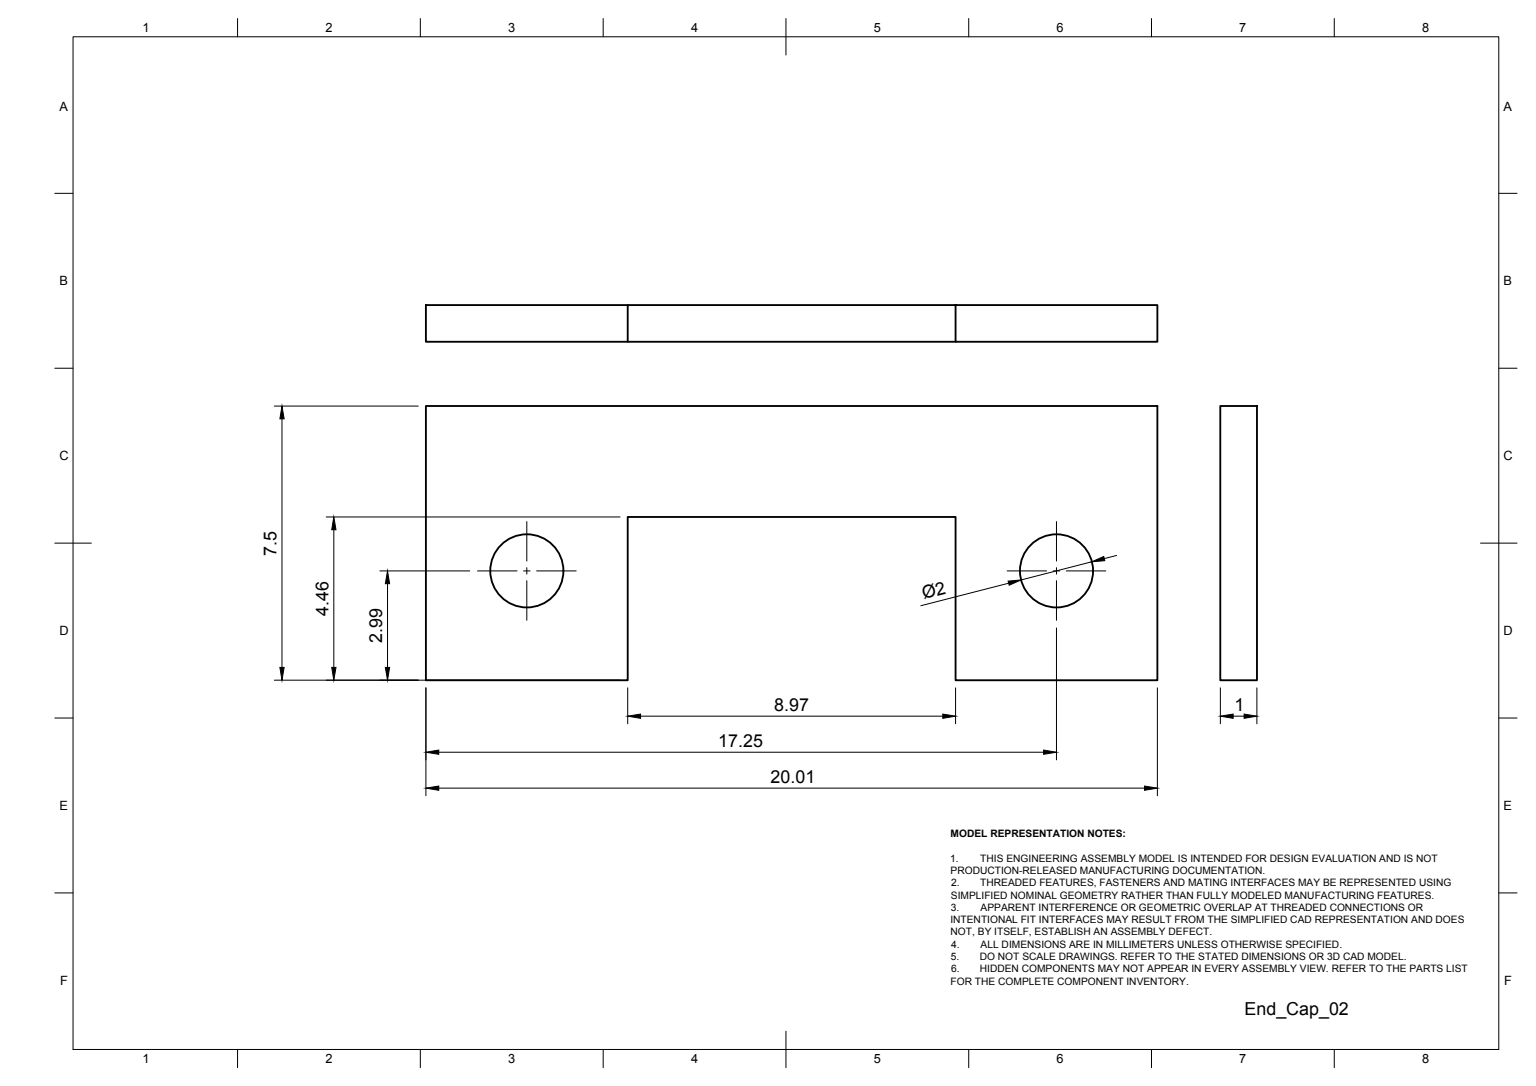
ISO-10303-21;
HEADER;
/* Generated by software containing ST-Developer
 * from STEP Tools, Inc. (www.steptools.com) 
 */

FILE_DESCRIPTION(
/* description */ (''),
/* implementation_level */ '2;1');

FILE_NAME(
/* name */ 'End_Cap_02.step',
/* time_stamp */ '2026-10-06T13:23:02-07:00',
/* author */ (''),
/* organization */ (''),
/* preprocessor_version */ 'ST-DEVELOPER v20.2',
/* originating_system */ 'Autodesk Translation Framework v15.15.0.0',
/* authorisation */ '');

FILE_SCHEMA (('AUTOMOTIVE_DESIGN { 1 0 10303 214 3 1 1 }'));
ENDSEC;

DATA;
#10=MECHANICAL_DESIGN_GEOMETRIC_PRESENTATION_REPRESENTATION('',(#79),#4994);
#59=SHAPE_REPRESENTATION_RELATIONSHIP('SRR','None',#5040,#69);
#69=ADVANCED_BREP_SHAPE_REPRESENTATION('',(#89),#4992);
#79=STYLED_ITEM('',(#5094),#89);
#89=MANIFOLD_SOLID_BREP('Body1',#2919);
#119=CYLINDRICAL_SURFACE('',#3269,1.);
#120=CYLINDRICAL_SURFACE('',#3272,1.);
#158=FACE_BOUND('',#681,.T.);
#159=FACE_BOUND('',#682,.T.);
#160=FACE_BOUND('',#684,.T.);
#161=FACE_BOUND('',#685,.T.);
#279=PLANE('',#3275);
#280=PLANE('',#3276);
#281=PLANE('',#3277);
#282=PLANE('',#3278);
#283=PLANE('',#3279);
#284=PLANE('',#3280);
#285=PLANE('',#3281);
#286=PLANE('',#3282);
#287=PLANE('',#3283);
#288=PLANE('',#3284);
#457=FACE_OUTER_BOUND('',#670,.T.);
#458=FACE_OUTER_BOUND('',#671,.T.);
#459=FACE_OUTER_BOUND('',#672,.T.);
#460=FACE_OUTER_BOUND('',#673,.T.);
#461=FACE_OUTER_BOUND('',#674,.T.);
#462=FACE_OUTER_BOUND('',#675,.T.);
#463=FACE_OUTER_BOUND('',#676,.T.);
#464=FACE_OUTER_BOUND('',#677,.T.);
#465=FACE_OUTER_BOUND('',#678,.T.);
#466=FACE_OUTER_BOUND('',#679,.T.);
#467=FACE_OUTER_BOUND('',#680,.T.);
#468=FACE_OUTER_BOUND('',#683,.T.);
#670=EDGE_LOOP('',(#2604,#2605,#2606,#2607));
#671=EDGE_LOOP('',(#2608,#2609,#2610,#2611));
#672=EDGE_LOOP('',(#2612,#2613,#2614,#2615));
#673=EDGE_LOOP('',(#2616,#2617,#2618,#2619));
#674=EDGE_LOOP('',(#2620,#2621,#2622,#2623));
#675=EDGE_LOOP('',(#2624,#2625,#2626,#2627));
#676=EDGE_LOOP('',(#2628,#2629,#2630,#2631));
#677=EDGE_LOOP('',(#2632,#2633,#2634,#2635));
#678=EDGE_LOOP('',(#2636,#2637,#2638,#2639));
#679=EDGE_LOOP('',(#2640,#2641,#2642,#2643));
#680=EDGE_LOOP('',(#2644,#2645,#2646,#2647,#2648,#2649,#2650,#2651));
#681=EDGE_LOOP('',(#2652));
#682=EDGE_LOOP('',(#2653));
#683=EDGE_LOOP('',(#2654,#2655,#2656,#2657,#2658,#2659,#2660,#2661));
#684=EDGE_LOOP('',(#2662));
#685=EDGE_LOOP('',(#2663));
#943=LINE('',#4840,#1236);
#944=LINE('',#4846,#1237);
#945=LINE('',#4851,#1238);
#946=LINE('',#4853,#1239);
#947=LINE('',#4855,#1240);
#948=LINE('',#4856,#1241);
#949=LINE('',#4859,#1242);
#950=LINE('',#4861,#1243);
#951=LINE('',#4862,#1244);
#952=LINE('',#4865,#1245);
#953=LINE('',#4867,#1246);
#954=LINE('',#4868,#1247);
#955=LINE('',#4871,#1248);
#956=LINE('',#4873,#1249);
#957=LINE('',#4874,#1250);
#958=LINE('',#4877,#1251);
#959=LINE('',#4879,#1252);
#960=LINE('',#4880,#1253);
#961=LINE('',#4883,#1254);
#962=LINE('',#4885,#1255);
#963=LINE('',#4886,#1256);
#964=LINE('',#4889,#1257);
#965=LINE('',#4891,#1258);
#966=LINE('',#4892,#1259);
#967=LINE('',#4894,#1260);
#968=LINE('',#4895,#1261);
#1236=VECTOR('',#4031,1.);
#1237=VECTOR('',#4038,1.);
#1238=VECTOR('',#4043,10.);
#1239=VECTOR('',#4044,10.);
#1240=VECTOR('',#4045,10.);
#1241=VECTOR('',#4046,10.);
#1242=VECTOR('',#4049,10.);
#1243=VECTOR('',#4050,10.);
#1244=VECTOR('',#4051,10.);
#1245=VECTOR('',#4054,10.);
#1246=VECTOR('',#4055,10.);
#1247=VECTOR('',#4056,10.);
#1248=VECTOR('',#4059,10.);
#1249=VECTOR('',#4060,10.);
#1250=VECTOR('',#4061,10.);
#1251=VECTOR('',#4064,10.);
#1252=VECTOR('',#4065,10.);
#1253=VECTOR('',#4066,10.);
#1254=VECTOR('',#4069,10.);
#1255=VECTOR('',#4070,10.);
#1256=VECTOR('',#4071,10.);
#1257=VECTOR('',#4074,10.);
#1258=VECTOR('',#4075,10.);
#1259=VECTOR('',#4076,10.);
#1260=VECTOR('',#4079,10.);
#1261=VECTOR('',#4080,10.);
#1361=CIRCLE('',#3270,1.);
#1362=CIRCLE('',#3271,1.);
#1363=CIRCLE('',#3273,1.);
#1364=CIRCLE('',#3274,1.);
#1562=VERTEX_POINT('',#4837);
#1563=VERTEX_POINT('',#4839);
#1564=VERTEX_POINT('',#4843);
#1565=VERTEX_POINT('',#4845);
#1566=VERTEX_POINT('',#4849);
#1567=VERTEX_POINT('',#4850);
#1568=VERTEX_POINT('',#4852);
#1569=VERTEX_POINT('',#4854);
#1570=VERTEX_POINT('',#4858);
#1571=VERTEX_POINT('',#4860);
#1572=VERTEX_POINT('',#4864);
#1573=VERTEX_POINT('',#4866);
#1574=VERTEX_POINT('',#4870);
#1575=VERTEX_POINT('',#4872);
#1576=VERTEX_POINT('',#4876);
#1577=VERTEX_POINT('',#4878);
#1578=VERTEX_POINT('',#4882);
#1579=VERTEX_POINT('',#4884);
#1580=VERTEX_POINT('',#4888);
#1581=VERTEX_POINT('',#4890);
#1916=EDGE_CURVE('',#1562,#1562,#1361,.T.);
#1917=EDGE_CURVE('',#1562,#1563,#943,.T.);
#1918=EDGE_CURVE('',#1563,#1563,#1362,.T.);
#1919=EDGE_CURVE('',#1564,#1564,#1363,.T.);
#1920=EDGE_CURVE('',#1564,#1565,#944,.T.);
#1921=EDGE_CURVE('',#1565,#1565,#1364,.T.);
#1922=EDGE_CURVE('',#1566,#1567,#945,.T.);
#1923=EDGE_CURVE('',#1566,#1568,#946,.T.);
#1924=EDGE_CURVE('',#1568,#1569,#947,.T.);
#1925=EDGE_CURVE('',#1567,#1569,#948,.T.);
#1926=EDGE_CURVE('',#1570,#1566,#949,.T.);
#1927=EDGE_CURVE('',#1570,#1571,#950,.T.);
#1928=EDGE_CURVE('',#1571,#1568,#951,.T.);
#1929=EDGE_CURVE('',#1572,#1570,#952,.T.);
#1930=EDGE_CURVE('',#1572,#1573,#953,.T.);
#1931=EDGE_CURVE('',#1573,#1571,#954,.T.);
#1932=EDGE_CURVE('',#1574,#1572,#955,.T.);
#1933=EDGE_CURVE('',#1574,#1575,#956,.T.);
#1934=EDGE_CURVE('',#1575,#1573,#957,.T.);
#1935=EDGE_CURVE('',#1576,#1574,#958,.T.);
#1936=EDGE_CURVE('',#1576,#1577,#959,.T.);
#1937=EDGE_CURVE('',#1577,#1575,#960,.T.);
#1938=EDGE_CURVE('',#1578,#1576,#961,.T.);
#1939=EDGE_CURVE('',#1578,#1579,#962,.T.);
#1940=EDGE_CURVE('',#1579,#1577,#963,.T.);
#1941=EDGE_CURVE('',#1580,#1578,#964,.T.);
#1942=EDGE_CURVE('',#1580,#1581,#965,.T.);
#1943=EDGE_CURVE('',#1581,#1579,#966,.T.);
#1944=EDGE_CURVE('',#1567,#1580,#967,.T.);
#1945=EDGE_CURVE('',#1569,#1581,#968,.T.);
#2604=ORIENTED_EDGE('',*,*,#1916,.T.);
#2605=ORIENTED_EDGE('',*,*,#1917,.T.);
#2606=ORIENTED_EDGE('',*,*,#1918,.T.);
#2607=ORIENTED_EDGE('',*,*,#1917,.F.);
#2608=ORIENTED_EDGE('',*,*,#1919,.T.);
#2609=ORIENTED_EDGE('',*,*,#1920,.T.);
#2610=ORIENTED_EDGE('',*,*,#1921,.T.);
#2611=ORIENTED_EDGE('',*,*,#1920,.F.);
#2612=ORIENTED_EDGE('',*,*,#1922,.F.);
#2613=ORIENTED_EDGE('',*,*,#1923,.T.);
#2614=ORIENTED_EDGE('',*,*,#1924,.T.);
#2615=ORIENTED_EDGE('',*,*,#1925,.F.);
#2616=ORIENTED_EDGE('',*,*,#1926,.F.);
#2617=ORIENTED_EDGE('',*,*,#1927,.T.);
#2618=ORIENTED_EDGE('',*,*,#1928,.T.);
#2619=ORIENTED_EDGE('',*,*,#1923,.F.);
#2620=ORIENTED_EDGE('',*,*,#1929,.F.);
#2621=ORIENTED_EDGE('',*,*,#1930,.T.);
#2622=ORIENTED_EDGE('',*,*,#1931,.T.);
#2623=ORIENTED_EDGE('',*,*,#1927,.F.);
#2624=ORIENTED_EDGE('',*,*,#1932,.F.);
#2625=ORIENTED_EDGE('',*,*,#1933,.T.);
#2626=ORIENTED_EDGE('',*,*,#1934,.T.);
#2627=ORIENTED_EDGE('',*,*,#1930,.F.);
#2628=ORIENTED_EDGE('',*,*,#1935,.F.);
#2629=ORIENTED_EDGE('',*,*,#1936,.T.);
#2630=ORIENTED_EDGE('',*,*,#1937,.T.);
#2631=ORIENTED_EDGE('',*,*,#1933,.F.);
#2632=ORIENTED_EDGE('',*,*,#1938,.F.);
#2633=ORIENTED_EDGE('',*,*,#1939,.T.);
#2634=ORIENTED_EDGE('',*,*,#1940,.T.);
#2635=ORIENTED_EDGE('',*,*,#1936,.F.);
#2636=ORIENTED_EDGE('',*,*,#1941,.F.);
#2637=ORIENTED_EDGE('',*,*,#1942,.T.);
#2638=ORIENTED_EDGE('',*,*,#1943,.T.);
#2639=ORIENTED_EDGE('',*,*,#1939,.F.);
#2640=ORIENTED_EDGE('',*,*,#1944,.F.);
#2641=ORIENTED_EDGE('',*,*,#1925,.T.);
#2642=ORIENTED_EDGE('',*,*,#1945,.T.);
#2643=ORIENTED_EDGE('',*,*,#1942,.F.);
#2644=ORIENTED_EDGE('',*,*,#1945,.F.);
#2645=ORIENTED_EDGE('',*,*,#1924,.F.);
#2646=ORIENTED_EDGE('',*,*,#1928,.F.);
#2647=ORIENTED_EDGE('',*,*,#1931,.F.);
#2648=ORIENTED_EDGE('',*,*,#1934,.F.);
#2649=ORIENTED_EDGE('',*,*,#1937,.F.);
#2650=ORIENTED_EDGE('',*,*,#1940,.F.);
#2651=ORIENTED_EDGE('',*,*,#1943,.F.);
#2652=ORIENTED_EDGE('',*,*,#1918,.F.);
#2653=ORIENTED_EDGE('',*,*,#1921,.F.);
#2654=ORIENTED_EDGE('',*,*,#1944,.T.);
#2655=ORIENTED_EDGE('',*,*,#1941,.T.);
#2656=ORIENTED_EDGE('',*,*,#1938,.T.);
#2657=ORIENTED_EDGE('',*,*,#1935,.T.);
#2658=ORIENTED_EDGE('',*,*,#1932,.T.);
#2659=ORIENTED_EDGE('',*,*,#1929,.T.);
#2660=ORIENTED_EDGE('',*,*,#1926,.T.);
#2661=ORIENTED_EDGE('',*,*,#1922,.T.);
#2662=ORIENTED_EDGE('',*,*,#1916,.F.);
#2663=ORIENTED_EDGE('',*,*,#1919,.F.);
#2887=ADVANCED_FACE('',(#457),#119,.F.);
#2888=ADVANCED_FACE('',(#458),#120,.F.);
#2889=ADVANCED_FACE('',(#459),#279,.F.);
#2890=ADVANCED_FACE('',(#460),#280,.F.);
#2891=ADVANCED_FACE('',(#461),#281,.F.);
#2892=ADVANCED_FACE('',(#462),#282,.F.);
#2893=ADVANCED_FACE('',(#463),#283,.F.);
#2894=ADVANCED_FACE('',(#464),#284,.F.);
#2895=ADVANCED_FACE('',(#465),#285,.F.);
#2896=ADVANCED_FACE('',(#466),#286,.F.);
#2897=ADVANCED_FACE('',(#467,#158,#159),#287,.F.);
#2898=ADVANCED_FACE('',(#468,#160,#161),#288,.T.);
#2919=CLOSED_SHELL('',(#2887,#2888,#2889,#2890,#2891,#2892,#2893,#2894,
#2895,#2896,#2897,#2898));
#3268=AXIS2_PLACEMENT_3D('',#4835,#4025,#4026);
#3269=AXIS2_PLACEMENT_3D('',#4836,#4027,#4028);
#3270=AXIS2_PLACEMENT_3D('',#4838,#4029,#4030);
#3271=AXIS2_PLACEMENT_3D('',#4841,#4032,#4033);
#3272=AXIS2_PLACEMENT_3D('',#4842,#4034,#4035);
#3273=AXIS2_PLACEMENT_3D('',#4844,#4036,#4037);
#3274=AXIS2_PLACEMENT_3D('',#4847,#4039,#4040);
#3275=AXIS2_PLACEMENT_3D('',#4848,#4041,#4042);
#3276=AXIS2_PLACEMENT_3D('',#4857,#4047,#4048);
#3277=AXIS2_PLACEMENT_3D('',#4863,#4052,#4053);
#3278=AXIS2_PLACEMENT_3D('',#4869,#4057,#4058);
#3279=AXIS2_PLACEMENT_3D('',#4875,#4062,#4063);
#3280=AXIS2_PLACEMENT_3D('',#4881,#4067,#4068);
#3281=AXIS2_PLACEMENT_3D('',#4887,#4072,#4073);
#3282=AXIS2_PLACEMENT_3D('',#4893,#4077,#4078);
#3283=AXIS2_PLACEMENT_3D('',#4896,#4081,#4082);
#3284=AXIS2_PLACEMENT_3D('',#4897,#4083,#4084);
#4025=DIRECTION('axis',(0.,0.,1.));
#4026=DIRECTION('refdir',(1.,0.,0.));
#4027=DIRECTION('center_axis',(-1.,0.,0.));
#4028=DIRECTION('ref_axis',(0.,1.,0.));
#4029=DIRECTION('center_axis',(1.,0.,0.));
#4030=DIRECTION('ref_axis',(0.,1.,0.));
#4031=DIRECTION('',(-1.,0.,0.));
#4032=DIRECTION('center_axis',(-1.,0.,0.));
#4033=DIRECTION('ref_axis',(0.,1.,0.));
#4034=DIRECTION('center_axis',(-1.,0.,0.));
#4035=DIRECTION('ref_axis',(0.,1.,0.));
#4036=DIRECTION('center_axis',(1.,0.,0.));
#4037=DIRECTION('ref_axis',(0.,1.,0.));
#4038=DIRECTION('',(-1.,0.,0.));
#4039=DIRECTION('center_axis',(-1.,0.,0.));
#4040=DIRECTION('ref_axis',(0.,1.,0.));
#4041=DIRECTION('center_axis',(0.,-1.,0.));
#4042=DIRECTION('ref_axis',(0.,0.,1.));
#4043=DIRECTION('',(0.,0.,1.));
#4044=DIRECTION('',(-1.,0.,0.));
#4045=DIRECTION('',(0.,0.,1.));
#4046=DIRECTION('',(-1.,0.,0.));
#4047=DIRECTION('center_axis',(0.,0.,1.));
#4048=DIRECTION('ref_axis',(0.,1.,0.));
#4049=DIRECTION('',(0.,1.,0.));
#4050=DIRECTION('',(-1.,0.,0.));
#4051=DIRECTION('',(0.,1.,0.));
#4052=DIRECTION('center_axis',(0.,1.,0.));
#4053=DIRECTION('ref_axis',(0.,0.,-1.));
#4054=DIRECTION('',(0.,0.,-1.));
#4055=DIRECTION('',(-1.,0.,0.));
#4056=DIRECTION('',(0.,0.,-1.));
#4057=DIRECTION('center_axis',(0.,0.,1.));
#4058=DIRECTION('ref_axis',(0.,1.,0.));
#4059=DIRECTION('',(0.,1.,0.));
#4060=DIRECTION('',(-1.,0.,0.));
#4061=DIRECTION('',(0.,1.,0.));
#4062=DIRECTION('center_axis',(0.,-1.,0.));
#4063=DIRECTION('ref_axis',(0.,0.,1.));
#4064=DIRECTION('',(0.,0.,1.));
#4065=DIRECTION('',(-1.,0.,0.));
#4066=DIRECTION('',(0.,0.,1.));
#4067=DIRECTION('center_axis',(0.,0.,1.));
#4068=DIRECTION('ref_axis',(0.,1.,0.));
#4069=DIRECTION('',(0.,1.,0.));
#4070=DIRECTION('',(-1.,0.,0.));
#4071=DIRECTION('',(0.,1.,0.));
#4072=DIRECTION('center_axis',(0.,1.,0.));
#4073=DIRECTION('ref_axis',(0.,0.,-1.));
#4074=DIRECTION('',(0.,0.,-1.));
#4075=DIRECTION('',(-1.,0.,0.));
#4076=DIRECTION('',(0.,0.,-1.));
#4077=DIRECTION('center_axis',(0.,0.,-1.));
#4078=DIRECTION('ref_axis',(0.,-1.,0.));
#4079=DIRECTION('',(0.,-1.,0.));
#4080=DIRECTION('',(0.,-1.,0.));
#4081=DIRECTION('center_axis',(1.,0.,0.));
#4082=DIRECTION('ref_axis',(0.,0.,-1.));
#4083=DIRECTION('center_axis',(1.,0.,0.));
#4084=DIRECTION('ref_axis',(0.,1.,0.));
#4835=CARTESIAN_POINT('',(0.,0.,0.));
#4836=CARTESIAN_POINT('Origin',(-14.5,7.24395366693103,1.75498192028357));
#4837=CARTESIAN_POINT('',(-13.5,6.24395366693103,1.75498192028357));
#4838=CARTESIAN_POINT('Origin',(-13.5,7.24395366693103,1.75498192028357));
#4839=CARTESIAN_POINT('',(-14.5,6.24395366693103,1.75498192028357));
#4840=CARTESIAN_POINT('',(-14.5,6.24395366693103,1.75498192028357));
#4841=CARTESIAN_POINT('Origin',(-14.5,7.24395366693103,1.75498192028357));
#4842=CARTESIAN_POINT('Origin',(-14.5,-7.24395366693103,1.75498192028357));
#4843=CARTESIAN_POINT('',(-13.5,-8.24395366693103,1.75498192028357));
#4844=CARTESIAN_POINT('Origin',(-13.5,-7.24395366693103,1.75498192028357));
#4845=CARTESIAN_POINT('',(-14.5,-8.24395366693103,1.75498192028357));
#4846=CARTESIAN_POINT('',(-14.5,-8.24395366693103,1.75498192028357));
#4847=CARTESIAN_POINT('Origin',(-14.5,-7.24395366693103,1.75498192028357));
#4848=CARTESIAN_POINT('Origin',(-13.5,10.0039433906299,-1.2346845122375));
#4849=CARTESIAN_POINT('',(-13.5,10.0039433906299,-1.2346845122375));
#4850=CARTESIAN_POINT('',(-13.5,10.0039433906299,6.26348125396711));
#4851=CARTESIAN_POINT('',(-13.5,10.0039433906299,-1.2346845122375));
#4852=CARTESIAN_POINT('',(-14.5,10.0039433906299,-1.2346845122375));
#4853=CARTESIAN_POINT('',(-13.5,10.0039433906299,-1.2346845122375));
#4854=CARTESIAN_POINT('',(-14.5,10.0039433906299,6.26348125396711));
#4855=CARTESIAN_POINT('',(-14.5,10.0039433906299,-1.2346845122375));
#4856=CARTESIAN_POINT('',(-13.5,10.0039433906299,6.26348125396711));
#4857=CARTESIAN_POINT('Origin',(-13.5,4.48396394323217,-1.2346845122375));
#4858=CARTESIAN_POINT('',(-13.5,4.48396394323217,-1.2346845122375));
#4859=CARTESIAN_POINT('',(-13.5,4.48396394323217,-1.2346845122375));
#4860=CARTESIAN_POINT('',(-14.5,4.48396394323217,-1.2346845122375));
#4861=CARTESIAN_POINT('',(-13.5,4.48396394323217,-1.2346845122375));
#4862=CARTESIAN_POINT('',(-14.5,4.48396394323217,-1.2346845122375));
#4863=CARTESIAN_POINT('Origin',(-13.5,4.48396394323217,3.23022961141938));
#4864=CARTESIAN_POINT('',(-13.5,4.48396394323217,3.23022961141938));
#4865=CARTESIAN_POINT('',(-13.5,4.48396394323217,3.23022961141938));
#4866=CARTESIAN_POINT('',(-14.5,4.48396394323217,3.23022961141938));
#4867=CARTESIAN_POINT('',(-13.5,4.48396394323217,3.23022961141938));
#4868=CARTESIAN_POINT('',(-14.5,4.48396394323217,3.23022961141938));
#4869=CARTESIAN_POINT('Origin',(-13.5,-4.48396394323217,3.23022961141938));
#4870=CARTESIAN_POINT('',(-13.5,-4.48396394323217,3.23022961141938));
#4871=CARTESIAN_POINT('',(-13.5,-4.48396394323217,3.23022961141938));
#4872=CARTESIAN_POINT('',(-14.5,-4.48396394323217,3.23022961141938));
#4873=CARTESIAN_POINT('',(-13.5,-4.48396394323217,3.23022961141938));
#4874=CARTESIAN_POINT('',(-14.5,-4.48396394323217,3.23022961141938));
#4875=CARTESIAN_POINT('Origin',(-13.5,-4.48396394323217,-1.2346845122375));
#4876=CARTESIAN_POINT('',(-13.5,-4.48396394323217,-1.2346845122375));
#4877=CARTESIAN_POINT('',(-13.5,-4.48396394323217,-1.2346845122375));
#4878=CARTESIAN_POINT('',(-14.5,-4.48396394323217,-1.2346845122375));
#4879=CARTESIAN_POINT('',(-13.5,-4.48396394323217,-1.2346845122375));
#4880=CARTESIAN_POINT('',(-14.5,-4.48396394323217,-1.2346845122375));
#4881=CARTESIAN_POINT('Origin',(-13.5,-10.0039433906299,-1.2346845122375));
#4882=CARTESIAN_POINT('',(-13.5,-10.0039433906299,-1.2346845122375));
#4883=CARTESIAN_POINT('',(-13.5,-10.0039433906299,-1.2346845122375));
#4884=CARTESIAN_POINT('',(-14.5,-10.0039433906299,-1.2346845122375));
#4885=CARTESIAN_POINT('',(-13.5,-10.0039433906299,-1.2346845122375));
#4886=CARTESIAN_POINT('',(-14.5,-10.0039433906299,-1.2346845122375));
#4887=CARTESIAN_POINT('Origin',(-13.5,-10.0039433906299,6.26348125396711));
#4888=CARTESIAN_POINT('',(-13.5,-10.0039433906299,6.26348125396711));
#4889=CARTESIAN_POINT('',(-13.5,-10.0039433906299,6.26348125396711));
#4890=CARTESIAN_POINT('',(-14.5,-10.0039433906299,6.26348125396711));
#4891=CARTESIAN_POINT('',(-13.5,-10.0039433906299,6.26348125396711));
#4892=CARTESIAN_POINT('',(-14.5,-10.0039433906299,6.26348125396711));
#4893=CARTESIAN_POINT('Origin',(-13.5,10.0039433906299,6.26348125396711));
#4894=CARTESIAN_POINT('',(-13.5,10.0039433906299,6.26348125396711));
#4895=CARTESIAN_POINT('',(-14.5,10.0039433906299,6.26348125396711));
#4896=CARTESIAN_POINT('Origin',(-14.5,0.,2.51439837086481));
#4897=CARTESIAN_POINT('Origin',(-13.5,0.,2.51439837086481));
#4980=UNCERTAINTY_MEASURE_WITH_UNIT(LENGTH_MEASURE(0.01),#4995,
'DISTANCE_ACCURACY_VALUE',
'Maximum model space distance between geometric entities at asserted c
onnectivities');
#4982=UNCERTAINTY_MEASURE_WITH_UNIT(LENGTH_MEASURE(0.01),#4995,
'DISTANCE_ACCURACY_VALUE',
'Maximum model space distance between geometric entities at asserted c
onnectivities');
#4992=(
GEOMETRIC_REPRESENTATION_CONTEXT(3)
GLOBAL_UNCERTAINTY_ASSIGNED_CONTEXT((#4980))
GLOBAL_UNIT_ASSIGNED_CONTEXT((#4995,#4997,#4998))
REPRESENTATION_CONTEXT('','3D')
);
#4994=(
GEOMETRIC_REPRESENTATION_CONTEXT(3)
GLOBAL_UNCERTAINTY_ASSIGNED_CONTEXT((#4982))
GLOBAL_UNIT_ASSIGNED_CONTEXT((#4995,#4997,#4998))
REPRESENTATION_CONTEXT('','3D')
);
#4995=(
LENGTH_UNIT()
NAMED_UNIT(*)
SI_UNIT(.MILLI.,.METRE.)
);
#4997=(
NAMED_UNIT(*)
PLANE_ANGLE_UNIT()
SI_UNIT($,.RADIAN.)
);
#4998=(
NAMED_UNIT(*)
SI_UNIT($,.STERADIAN.)
SOLID_ANGLE_UNIT()
);
#5008=SHAPE_DEFINITION_REPRESENTATION(#5019,#5040);
#5019=PRODUCT_DEFINITION_SHAPE('',$,#5052);
#5040=SHAPE_REPRESENTATION('',(#3268),#4992);
#5042=PRODUCT_DEFINITION_CONTEXT('part definition',#5077,'design');
#5052=PRODUCT_DEFINITION('End_Cap_02','End_Cap_02',#5063,#5042);
#5063=PRODUCT_DEFINITION_FORMATION('',$,#5088);
#5077=APPLICATION_CONTEXT(
'Core Data for Automotive Mechanical Design Process');
#5078=PRODUCT_CONTEXT('part definition',#5077,'mechanical');
#5088=PRODUCT('End_Cap_02','End_Cap_02',$,(#5078));
#5094=PRESENTATION_STYLE_ASSIGNMENT((#5099));
#5099=SURFACE_STYLE_USAGE(.BOTH.,#5104);
#5104=SURFACE_SIDE_STYLE('',(#5109));
#5109=SURFACE_STYLE_FILL_AREA(#5114);
#5114=FILL_AREA_STYLE('Opaque(196,0,0)',(#5119));
#5119=FILL_AREA_STYLE_COLOUR('Opaque(196,0,0)',#5124);
#5124=COLOUR_RGB('Opaque(196,0,0)', 0.66274510, 0.83137255, 0.94901961);
ENDSEC;
END-ISO-10303-21;
